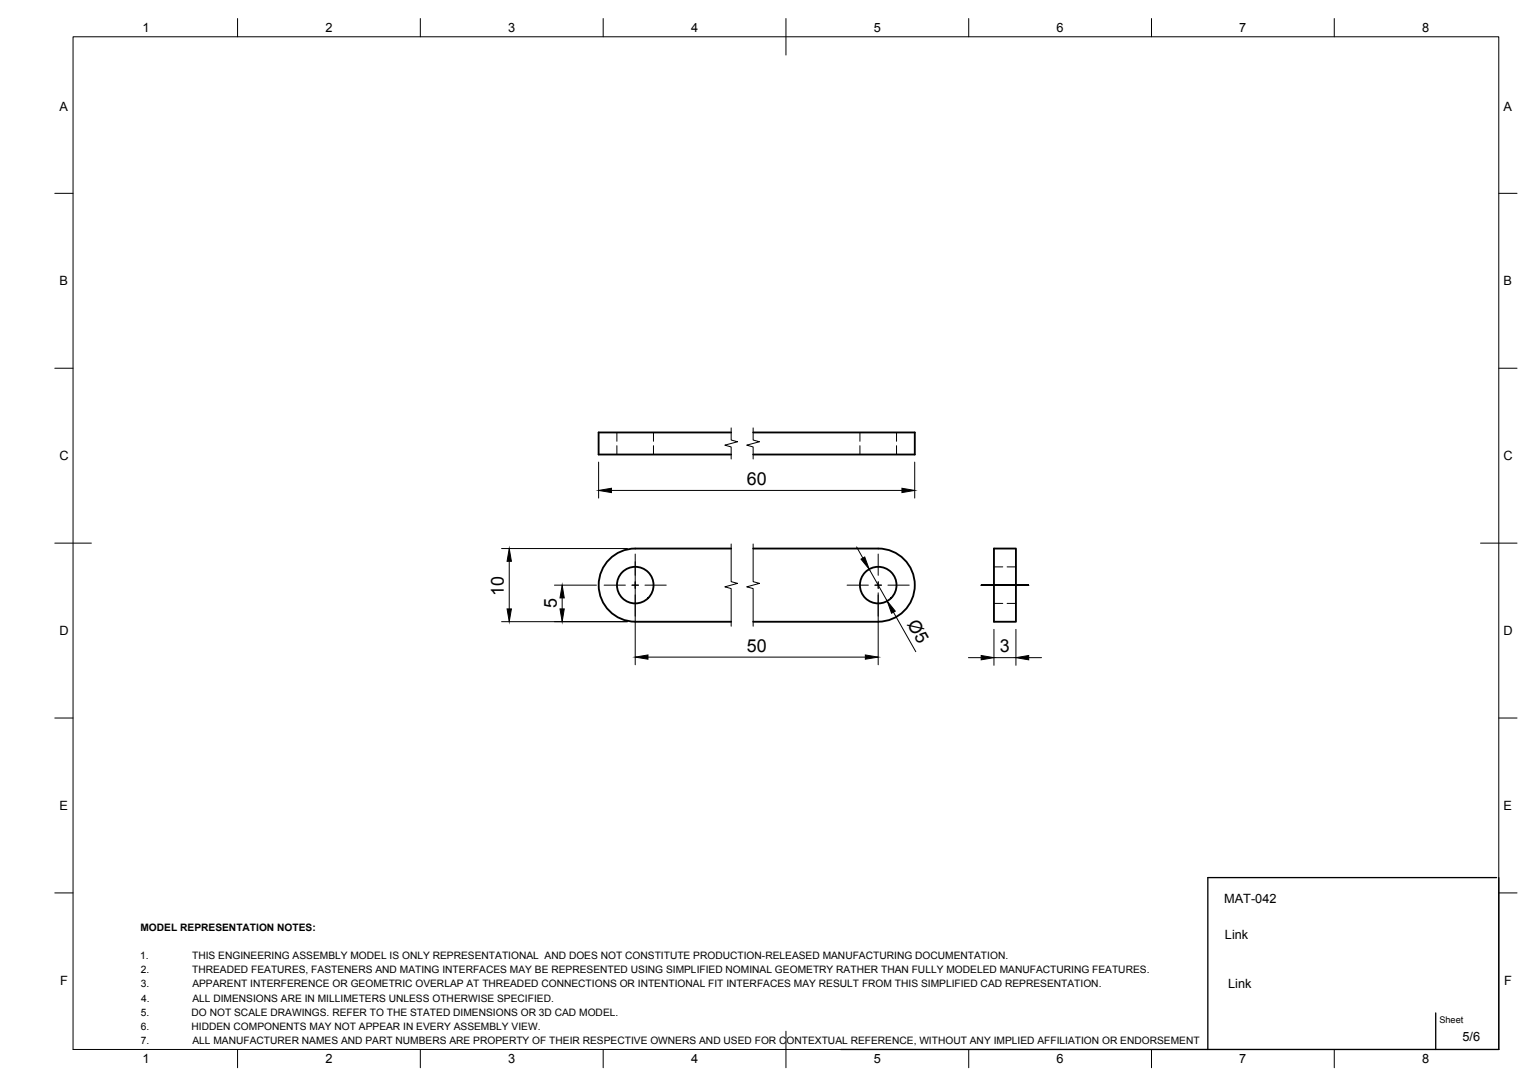
ISO-10303-21;
HEADER;
/* Generated by software containing ST-Developer
 * from STEP Tools, Inc. (www.steptools.com) 
 */

FILE_DESCRIPTION(
/* description */ ('STEP AP214'),
/* implementation_level */ '2;1');

FILE_NAME(
/* name */ 'Link.step',
/* time_stamp */ '2026-11-14T22:03:06-08:00',
/* author */ (''),
/* organization */ (''),
/* preprocessor_version */ 'ST-DEVELOPER v20.2',
/* originating_system */ 'Autodesk Translation Framework v15.17.0.0',
/* authorisation */ '');

FILE_SCHEMA (('AUTOMOTIVE_DESIGN { 1 0 10303 214 3 1 1 }'));
ENDSEC;

DATA;
#10=MECHANICAL_DESIGN_GEOMETRIC_PRESENTATION_REPRESENTATION('',(#310),#12966);
#290=SHAPE_REPRESENTATION_RELATIONSHIP('SRR','None',#13028,#298);
#298=ADVANCED_BREP_SHAPE_REPRESENTATION('',(#322),#12961);
#310=STYLED_ITEM('',(#13077),#322);
#322=MANIFOLD_SOLID_BREP('Body1',#5585);
#373=FACE_BOUND('',#1129,.T.);
#374=FACE_BOUND('',#1130,.T.);
#375=FACE_BOUND('',#1132,.T.);
#376=FACE_BOUND('',#1133,.T.);
#486=PLANE('',#6033);
#487=PLANE('',#6036);
#488=PLANE('',#6040);
#489=PLANE('',#6042);
#769=FACE_OUTER_BOUND('',#1126,.T.);
#770=FACE_OUTER_BOUND('',#1127,.T.);
#771=FACE_OUTER_BOUND('',#1128,.T.);
#772=FACE_OUTER_BOUND('',#1131,.T.);
#773=FACE_OUTER_BOUND('',#1134,.T.);
#774=FACE_OUTER_BOUND('',#1135,.T.);
#775=FACE_OUTER_BOUND('',#1136,.T.);
#776=FACE_OUTER_BOUND('',#1137,.T.);
#1126=EDGE_LOOP('',(#4801,#4802,#4803,#4804));
#1127=EDGE_LOOP('',(#4805,#4806,#4807,#4808));
#1128=EDGE_LOOP('',(#4809,#4810,#4811,#4812));
#1129=EDGE_LOOP('',(#4813));
#1130=EDGE_LOOP('',(#4814));
#1131=EDGE_LOOP('',(#4815,#4816,#4817,#4818));
#1132=EDGE_LOOP('',(#4819));
#1133=EDGE_LOOP('',(#4820));
#1134=EDGE_LOOP('',(#4821,#4822,#4823,#4824));
#1135=EDGE_LOOP('',(#4825,#4826,#4827,#4828));
#1136=EDGE_LOOP('',(#4829,#4830,#4831,#4832));
#1137=EDGE_LOOP('',(#4833,#4834,#4835,#4836));
#1569=LINE('',#12518,#2026);
#1570=LINE('',#12524,#2027);
#1571=LINE('',#12531,#2028);
#1572=LINE('',#12534,#2029);
#1573=LINE('',#12540,#2030);
#1574=LINE('',#12543,#2031);
#1575=LINE('',#12545,#2032);
#1576=LINE('',#12546,#2033);
#1577=LINE('',#12548,#2034);
#1578=LINE('',#12550,#2035);
#2026=VECTOR('',#7257,2.5);
#2027=VECTOR('',#7264,2.5);
#2028=VECTOR('',#7271,1000.);
#2029=VECTOR('',#7274,1000.);
#2030=VECTOR('',#7279,1000.);
#2031=VECTOR('',#7282,1000.);
#2032=VECTOR('',#7285,1000.);
#2033=VECTOR('',#7286,1000.);
#2034=VECTOR('',#7289,1000.);
#2035=VECTOR('',#7292,1000.);
#2312=CIRCLE('',#6028,2.5);
#2313=CIRCLE('',#6029,2.5);
#2314=CIRCLE('',#6031,2.5);
#2315=CIRCLE('',#6032,2.5);
#2316=CIRCLE('',#6034,5.);
#2317=CIRCLE('',#6035,5.);
#2318=CIRCLE('',#6037,5.);
#2319=CIRCLE('',#6038,5.);
#2762=VERTEX_POINT('',#12515);
#2763=VERTEX_POINT('',#12517);
#2764=VERTEX_POINT('',#12521);
#2765=VERTEX_POINT('',#12523);
#2766=VERTEX_POINT('',#12527);
#2767=VERTEX_POINT('',#12528);
#2768=VERTEX_POINT('',#12530);
#2769=VERTEX_POINT('',#12532);
#2770=VERTEX_POINT('',#12536);
#2771=VERTEX_POINT('',#12537);
#2772=VERTEX_POINT('',#12539);
#2773=VERTEX_POINT('',#12541);
#3457=EDGE_CURVE('',#2762,#2762,#2312,.T.);
#3458=EDGE_CURVE('',#2762,#2763,#1569,.T.);
#3459=EDGE_CURVE('',#2763,#2763,#2313,.T.);
#3460=EDGE_CURVE('',#2764,#2764,#2314,.T.);
#3461=EDGE_CURVE('',#2764,#2765,#1570,.T.);
#3462=EDGE_CURVE('',#2765,#2765,#2315,.T.);
#3463=EDGE_CURVE('',#2766,#2767,#2316,.T.);
#3464=EDGE_CURVE('',#2767,#2768,#1571,.T.);
#3465=EDGE_CURVE('',#2768,#2769,#2317,.T.);
#3466=EDGE_CURVE('',#2769,#2766,#1572,.T.);
#3467=EDGE_CURVE('',#2770,#2771,#2318,.T.);
#3468=EDGE_CURVE('',#2772,#2770,#1573,.T.);
#3469=EDGE_CURVE('',#2773,#2772,#2319,.T.);
#3470=EDGE_CURVE('',#2771,#2773,#1574,.T.);
#3471=EDGE_CURVE('',#2767,#2771,#1575,.T.);
#3472=EDGE_CURVE('',#2766,#2770,#1576,.T.);
#3473=EDGE_CURVE('',#2768,#2773,#1577,.T.);
#3474=EDGE_CURVE('',#2769,#2772,#1578,.T.);
#4801=ORIENTED_EDGE('',*,*,#3457,.T.);
#4802=ORIENTED_EDGE('',*,*,#3458,.T.);
#4803=ORIENTED_EDGE('',*,*,#3459,.F.);
#4804=ORIENTED_EDGE('',*,*,#3458,.F.);
#4805=ORIENTED_EDGE('',*,*,#3460,.T.);
#4806=ORIENTED_EDGE('',*,*,#3461,.T.);
#4807=ORIENTED_EDGE('',*,*,#3462,.F.);
#4808=ORIENTED_EDGE('',*,*,#3461,.F.);
#4809=ORIENTED_EDGE('',*,*,#3463,.T.);
#4810=ORIENTED_EDGE('',*,*,#3464,.T.);
#4811=ORIENTED_EDGE('',*,*,#3465,.T.);
#4812=ORIENTED_EDGE('',*,*,#3466,.T.);
#4813=ORIENTED_EDGE('',*,*,#3457,.F.);
#4814=ORIENTED_EDGE('',*,*,#3460,.F.);
#4815=ORIENTED_EDGE('',*,*,#3467,.F.);
#4816=ORIENTED_EDGE('',*,*,#3468,.F.);
#4817=ORIENTED_EDGE('',*,*,#3469,.F.);
#4818=ORIENTED_EDGE('',*,*,#3470,.F.);
#4819=ORIENTED_EDGE('',*,*,#3459,.T.);
#4820=ORIENTED_EDGE('',*,*,#3462,.T.);
#4821=ORIENTED_EDGE('',*,*,#3467,.T.);
#4822=ORIENTED_EDGE('',*,*,#3471,.F.);
#4823=ORIENTED_EDGE('',*,*,#3463,.F.);
#4824=ORIENTED_EDGE('',*,*,#3472,.T.);
#4825=ORIENTED_EDGE('',*,*,#3470,.T.);
#4826=ORIENTED_EDGE('',*,*,#3473,.F.);
#4827=ORIENTED_EDGE('',*,*,#3464,.F.);
#4828=ORIENTED_EDGE('',*,*,#3471,.T.);
#4829=ORIENTED_EDGE('',*,*,#3469,.T.);
#4830=ORIENTED_EDGE('',*,*,#3474,.F.);
#4831=ORIENTED_EDGE('',*,*,#3465,.F.);
#4832=ORIENTED_EDGE('',*,*,#3473,.T.);
#4833=ORIENTED_EDGE('',*,*,#3468,.T.);
#4834=ORIENTED_EDGE('',*,*,#3472,.F.);
#4835=ORIENTED_EDGE('',*,*,#3466,.F.);
#4836=ORIENTED_EDGE('',*,*,#3474,.T.);
#5255=CYLINDRICAL_SURFACE('',#6027,2.5);
#5256=CYLINDRICAL_SURFACE('',#6030,2.5);
#5257=CYLINDRICAL_SURFACE('',#6039,5.);
#5258=CYLINDRICAL_SURFACE('',#6041,5.);
#5486=ADVANCED_FACE('',(#769),#5255,.F.);
#5487=ADVANCED_FACE('',(#770),#5256,.F.);
#5488=ADVANCED_FACE('',(#771,#373,#374),#486,.T.);
#5489=ADVANCED_FACE('',(#772,#375,#376),#487,.F.);
#5490=ADVANCED_FACE('',(#773),#5257,.T.);
#5491=ADVANCED_FACE('',(#774),#488,.F.);
#5492=ADVANCED_FACE('',(#775),#5258,.T.);
#5493=ADVANCED_FACE('',(#776),#489,.F.);
#5585=CLOSED_SHELL('',(#5486,#5487,#5488,#5489,#5490,#5491,#5492,#5493));
#6026=AXIS2_PLACEMENT_3D('',#12513,#7251,#7252);
#6027=AXIS2_PLACEMENT_3D('',#12514,#7253,#7254);
#6028=AXIS2_PLACEMENT_3D('',#12516,#7255,#7256);
#6029=AXIS2_PLACEMENT_3D('',#12519,#7258,#7259);
#6030=AXIS2_PLACEMENT_3D('',#12520,#7260,#7261);
#6031=AXIS2_PLACEMENT_3D('',#12522,#7262,#7263);
#6032=AXIS2_PLACEMENT_3D('',#12525,#7265,#7266);
#6033=AXIS2_PLACEMENT_3D('',#12526,#7267,#7268);
#6034=AXIS2_PLACEMENT_3D('',#12529,#7269,#7270);
#6035=AXIS2_PLACEMENT_3D('',#12533,#7272,#7273);
#6036=AXIS2_PLACEMENT_3D('',#12535,#7275,#7276);
#6037=AXIS2_PLACEMENT_3D('',#12538,#7277,#7278);
#6038=AXIS2_PLACEMENT_3D('',#12542,#7280,#7281);
#6039=AXIS2_PLACEMENT_3D('',#12544,#7283,#7284);
#6040=AXIS2_PLACEMENT_3D('',#12547,#7287,#7288);
#6041=AXIS2_PLACEMENT_3D('',#12549,#7290,#7291);
#6042=AXIS2_PLACEMENT_3D('',#12551,#7293,#7294);
#7251=DIRECTION('axis',(0.,0.,1.));
#7252=DIRECTION('refdir',(1.,0.,0.));
#7253=DIRECTION('center_axis',(0.,-1.,0.));
#7254=DIRECTION('ref_axis',(0.,0.,-1.));
#7255=DIRECTION('center_axis',(0.,1.,0.));
#7256=DIRECTION('ref_axis',(0.,0.,1.));
#7257=DIRECTION('',(0.,-1.,0.));
#7258=DIRECTION('center_axis',(0.,1.,0.));
#7259=DIRECTION('ref_axis',(0.,0.,1.));
#7260=DIRECTION('center_axis',(0.,-1.,0.));
#7261=DIRECTION('ref_axis',(0.,0.,-1.));
#7262=DIRECTION('center_axis',(0.,1.,0.));
#7263=DIRECTION('ref_axis',(0.,0.,1.));
#7264=DIRECTION('',(0.,-1.,0.));
#7265=DIRECTION('center_axis',(0.,1.,0.));
#7266=DIRECTION('ref_axis',(0.,0.,1.));
#7267=DIRECTION('center_axis',(0.,1.,0.));
#7268=DIRECTION('ref_axis',(0.,0.,1.));
#7269=DIRECTION('center_axis',(0.,1.,0.));
#7270=DIRECTION('ref_axis',(0.,0.,1.));
#7271=DIRECTION('',(1.,0.,-1.90819582357449E-16));
#7272=DIRECTION('center_axis',(0.,1.,0.));
#7273=DIRECTION('ref_axis',(0.,0.,1.));
#7274=DIRECTION('',(-1.,0.,1.90819582357449E-16));
#7275=DIRECTION('center_axis',(0.,1.,0.));
#7276=DIRECTION('ref_axis',(0.,0.,1.));
#7277=DIRECTION('center_axis',(0.,1.,0.));
#7278=DIRECTION('ref_axis',(0.,0.,1.));
#7279=DIRECTION('',(-1.,0.,1.90819582357449E-16));
#7280=DIRECTION('center_axis',(0.,1.,0.));
#7281=DIRECTION('ref_axis',(0.,0.,1.));
#7282=DIRECTION('',(1.,0.,-1.90819582357449E-16));
#7283=DIRECTION('center_axis',(0.,-1.,0.));
#7284=DIRECTION('ref_axis',(0.,0.,-1.));
#7285=DIRECTION('',(0.,-1.,0.));
#7286=DIRECTION('',(0.,-1.,0.));
#7287=DIRECTION('center_axis',(-1.90819582357449E-16,0.,-1.));
#7288=DIRECTION('ref_axis',(-1.,0.,1.90819582357449E-16));
#7289=DIRECTION('',(0.,-1.,0.));
#7290=DIRECTION('center_axis',(0.,-1.,0.));
#7291=DIRECTION('ref_axis',(0.,0.,-1.));
#7292=DIRECTION('',(0.,-1.,0.));
#7293=DIRECTION('center_axis',(1.90819582357449E-16,0.,1.));
#7294=DIRECTION('ref_axis',(1.,0.,-1.90819582357449E-16));
#12513=CARTESIAN_POINT('',(0.,0.,0.));
#12514=CARTESIAN_POINT('Origin',(25.,3.,-9.18485099360515E-15));
#12515=CARTESIAN_POINT('',(25.,3.,2.49999999999999));
#12516=CARTESIAN_POINT('Origin',(25.,3.,-9.18485099360515E-15));
#12517=CARTESIAN_POINT('',(25.,0.,2.49999999999999));
#12518=CARTESIAN_POINT('',(25.,3.,2.49999999999999));
#12519=CARTESIAN_POINT('Origin',(25.,0.,-9.18485099360515E-15));
#12520=CARTESIAN_POINT('Origin',(-25.,3.,0.));
#12521=CARTESIAN_POINT('',(-25.,3.,2.5));
#12522=CARTESIAN_POINT('Origin',(-25.,3.,0.));
#12523=CARTESIAN_POINT('',(-25.,0.,2.5));
#12524=CARTESIAN_POINT('',(-25.,3.,2.5));
#12525=CARTESIAN_POINT('Origin',(-25.,0.,0.));
#12526=CARTESIAN_POINT('Origin',(-25.,3.,0.));
#12527=CARTESIAN_POINT('',(-25.,3.,-5.));
#12528=CARTESIAN_POINT('',(-25.,3.,5.));
#12529=CARTESIAN_POINT('Origin',(-25.,3.,0.));
#12530=CARTESIAN_POINT('',(25.,3.,4.99999999999999));
#12531=CARTESIAN_POINT('',(-25.,3.,5.));
#12532=CARTESIAN_POINT('',(25.,3.,-5.00000000000001));
#12533=CARTESIAN_POINT('Origin',(25.,3.,-9.18485099360515E-15));
#12534=CARTESIAN_POINT('',(-25.,3.,-5.));
#12535=CARTESIAN_POINT('Origin',(-25.,0.,0.));
#12536=CARTESIAN_POINT('',(-25.,0.,-5.));
#12537=CARTESIAN_POINT('',(-25.,0.,5.));
#12538=CARTESIAN_POINT('Origin',(-25.,0.,0.));
#12539=CARTESIAN_POINT('',(25.,0.,-5.00000000000001));
#12540=CARTESIAN_POINT('',(-25.,0.,-5.));
#12541=CARTESIAN_POINT('',(25.,0.,4.99999999999999));
#12542=CARTESIAN_POINT('Origin',(25.,0.,-9.18485099360515E-15));
#12543=CARTESIAN_POINT('',(-25.,0.,5.));
#12544=CARTESIAN_POINT('Origin',(-25.,3.,0.));
#12545=CARTESIAN_POINT('',(-25.,3.,5.));
#12546=CARTESIAN_POINT('',(-25.,3.,-5.));
#12547=CARTESIAN_POINT('Origin',(-25.,3.,5.));
#12548=CARTESIAN_POINT('',(25.,3.,4.99999999999999));
#12549=CARTESIAN_POINT('Origin',(25.,3.,-9.18485099360515E-15));
#12550=CARTESIAN_POINT('',(25.,3.,-5.00000000000001));
#12551=CARTESIAN_POINT('Origin',(-25.,3.,-5.));
#12951=UNCERTAINTY_MEASURE_WITH_UNIT(LENGTH_MEASURE(0.01),#12967,
'DISTANCE_ACCURACY_VALUE',
'Maximum model space distance between geometric entities at asserted c
onnectivities');
#12956=UNCERTAINTY_MEASURE_WITH_UNIT(LENGTH_MEASURE(0.01),#12967,
'DISTANCE_ACCURACY_VALUE',
'Maximum model space distance between geometric entities at asserted c
onnectivities');
#12961=(
GEOMETRIC_REPRESENTATION_CONTEXT(3)
GLOBAL_UNCERTAINTY_ASSIGNED_CONTEXT((#12951))
GLOBAL_UNIT_ASSIGNED_CONTEXT((#12967,#12969,#12970))
REPRESENTATION_CONTEXT('','3D')
);
#12966=(
GEOMETRIC_REPRESENTATION_CONTEXT(3)
GLOBAL_UNCERTAINTY_ASSIGNED_CONTEXT((#12956))
GLOBAL_UNIT_ASSIGNED_CONTEXT((#12967,#12969,#12970))
REPRESENTATION_CONTEXT('','3D')
);
#12967=(
LENGTH_UNIT()
NAMED_UNIT(*)
SI_UNIT(.MILLI.,.METRE.)
);
#12969=(
NAMED_UNIT(*)
PLANE_ANGLE_UNIT()
SI_UNIT($,.RADIAN.)
);
#12970=(
NAMED_UNIT(*)
SI_UNIT($,.STERADIAN.)
SOLID_ANGLE_UNIT()
);
#12975=SHAPE_DEFINITION_REPRESENTATION(#12984,#13028);
#12984=PRODUCT_DEFINITION_SHAPE('',$,#13038);
#13028=SHAPE_REPRESENTATION('',(#6026),#12961);
#13033=PRODUCT_DEFINITION_CONTEXT('part definition',#13062,'design');
#13038=PRODUCT_DEFINITION('Link','Link',#13047,#13033);
#13047=PRODUCT_DEFINITION_FORMATION('',$,#13068);
#13062=APPLICATION_CONTEXT(
'Core Data for Automotive Mechanical Design Process');
#13063=PRODUCT_CONTEXT('part definition',#13062,'mechanical');
#13068=PRODUCT('Link','Link',$,(#13063));
#13077=PRESENTATION_STYLE_ASSIGNMENT((#13082));
#13082=SURFACE_STYLE_USAGE(.BOTH.,#13087);
#13087=SURFACE_SIDE_STYLE('',(#13092));
#13092=SURFACE_STYLE_FILL_AREA(#13097);
#13097=FILL_AREA_STYLE('Opaque(61,176,222)',(#13102));
#13102=FILL_AREA_STYLE_COLOUR('Opaque(61,176,222)',#13107);
#13107=COLOUR_RGB('Opaque(61,176,222)',0.23921568627451,0.690196078431373,
0.870588235294118);
ENDSEC;
END-ISO-10303-21;
